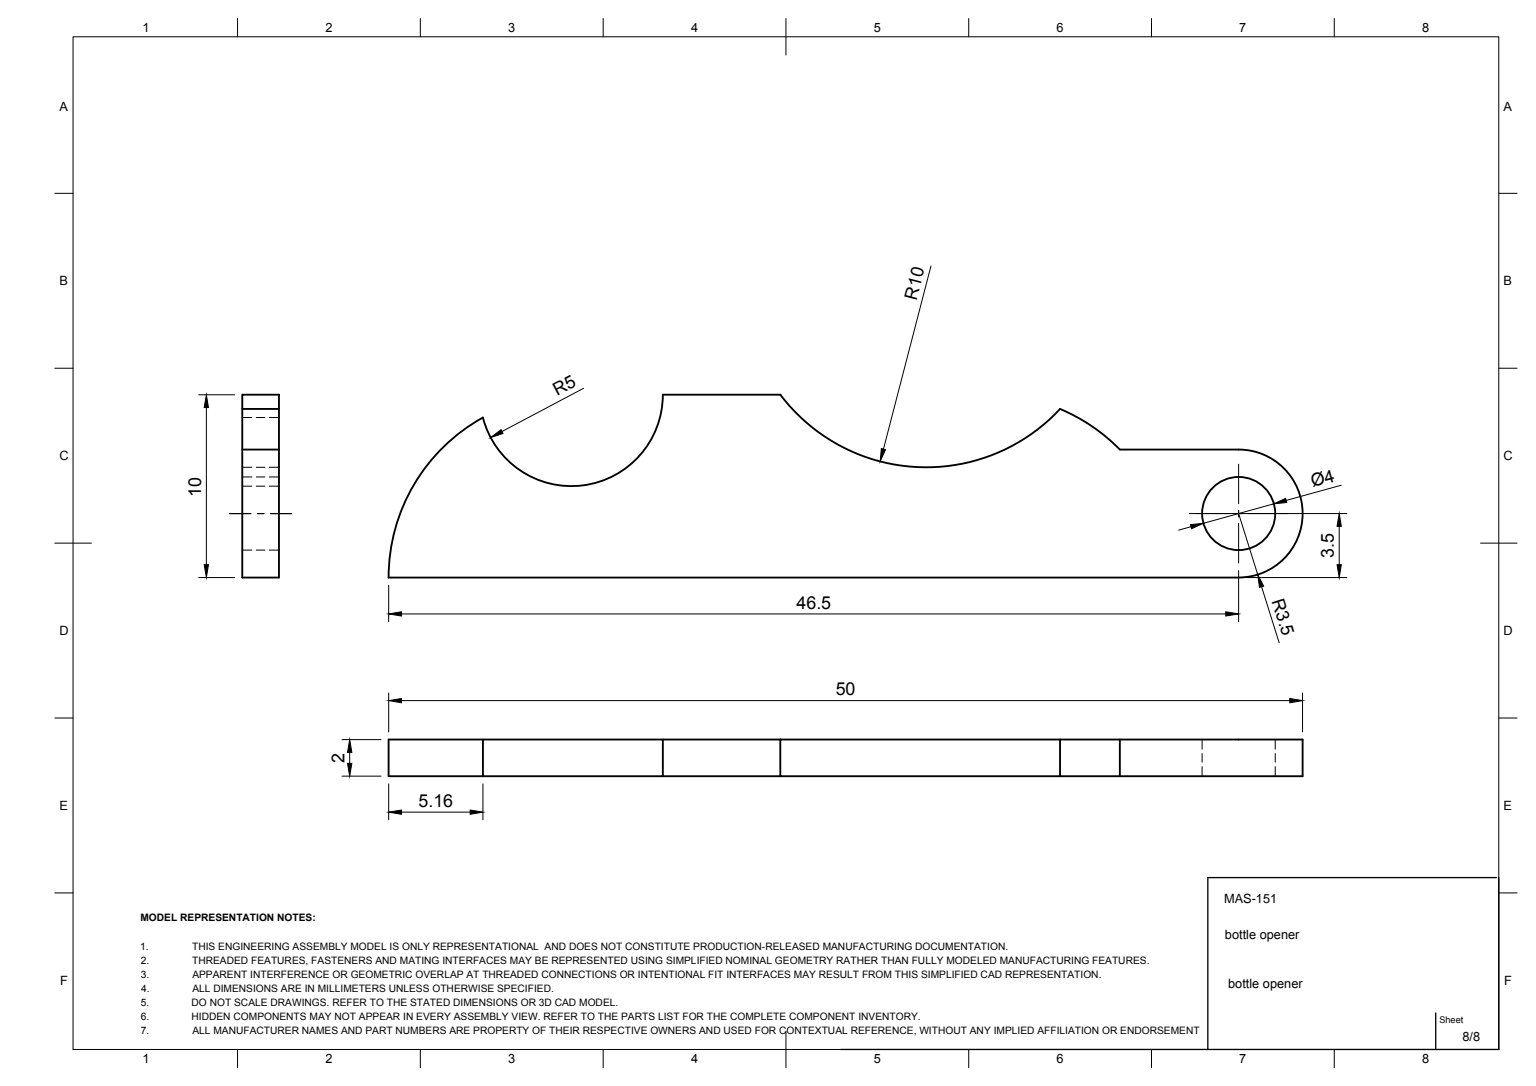
ISO-10303-21;
HEADER;
/* Generated by software containing ST-Developer
 * from STEP Tools, Inc. (www.steptools.com) 
 */

FILE_DESCRIPTION(
/* description */ ('STEP AP214'),
/* implementation_level */ '2;1');

FILE_NAME(
/* name */ 'bottle opener.step',
/* time_stamp */ '2026-11-04T19:14:12-08:00',
/* author */ (''),
/* organization */ (''),
/* preprocessor_version */ 'ST-DEVELOPER v20.2',
/* originating_system */ 'Autodesk Translation Framework v15.17.0.0',
/* authorisation */ '');

FILE_SCHEMA (('AUTOMOTIVE_DESIGN { 1 0 10303 214 3 1 1 }'));
ENDSEC;

DATA;
#10=MECHANICAL_DESIGN_GEOMETRIC_PRESENTATION_REPRESENTATION('',(#104),#5990);
#90=SHAPE_REPRESENTATION_RELATIONSHIP('SRR','None',#6026,#97);
#97=ADVANCED_BREP_SHAPE_REPRESENTATION('',(#111),#5988);
#104=STYLED_ITEM('',(#6068),#111);
#111=MANIFOLD_SOLID_BREP('Body1',#3274);
#133=FACE_BOUND('',#604,.T.);
#134=FACE_BOUND('',#606,.T.);
#233=PLANE('',#3648);
#234=PLANE('',#3652);
#235=PLANE('',#3656);
#236=PLANE('',#3657);
#237=PLANE('',#3658);
#402=FACE_OUTER_BOUND('',#600,.T.);
#403=FACE_OUTER_BOUND('',#601,.T.);
#404=FACE_OUTER_BOUND('',#602,.T.);
#405=FACE_OUTER_BOUND('',#603,.T.);
#406=FACE_OUTER_BOUND('',#605,.T.);
#407=FACE_OUTER_BOUND('',#607,.T.);
#408=FACE_OUTER_BOUND('',#608,.T.);
#409=FACE_OUTER_BOUND('',#609,.T.);
#410=FACE_OUTER_BOUND('',#610,.T.);
#411=FACE_OUTER_BOUND('',#611,.T.);
#412=FACE_OUTER_BOUND('',#612,.T.);
#600=EDGE_LOOP('',(#2956,#2957,#2958,#2959));
#601=EDGE_LOOP('',(#2960,#2961,#2962,#2963));
#602=EDGE_LOOP('',(#2964,#2965,#2966,#2967));
#603=EDGE_LOOP('',(#2968,#2969,#2970,#2971,#2972,#2973,#2974,#2975));
#604=EDGE_LOOP('',(#2976));
#605=EDGE_LOOP('',(#2977,#2978,#2979,#2980,#2981,#2982,#2983,#2984));
#606=EDGE_LOOP('',(#2985));
#607=EDGE_LOOP('',(#2986,#2987,#2988,#2989));
#608=EDGE_LOOP('',(#2990,#2991,#2992,#2993));
#609=EDGE_LOOP('',(#2994,#2995,#2996,#2997));
#610=EDGE_LOOP('',(#2998,#2999,#3000,#3001));
#611=EDGE_LOOP('',(#3002,#3003,#3004,#3005));
#612=EDGE_LOOP('',(#3006,#3007,#3008,#3009));
#907=LINE('',#5889,#1210);
#908=LINE('',#5896,#1211);
#909=LINE('',#5899,#1212);
#910=LINE('',#5905,#1213);
#911=LINE('',#5908,#1214);
#912=LINE('',#5912,#1215);
#913=LINE('',#5916,#1216);
#914=LINE('',#5918,#1217);
#915=LINE('',#5925,#1218);
#916=LINE('',#5927,#1219);
#917=LINE('',#5930,#1220);
#918=LINE('',#5933,#1221);
#919=LINE('',#5934,#1222);
#920=LINE('',#5936,#1223);
#921=LINE('',#5937,#1224);
#1210=VECTOR('',#4544,2.);
#1211=VECTOR('',#4551,1000.);
#1212=VECTOR('',#4554,1000.);
#1213=VECTOR('',#4559,1000.);
#1214=VECTOR('',#4562,1000.);
#1215=VECTOR('',#4565,1000.);
#1216=VECTOR('',#4568,1000.);
#1217=VECTOR('',#4571,1000.);
#1218=VECTOR('',#4578,1000.);
#1219=VECTOR('',#4581,1000.);
#1220=VECTOR('',#4584,1000.);
#1221=VECTOR('',#4589,1000.);
#1222=VECTOR('',#4590,1000.);
#1223=VECTOR('',#4593,1000.);
#1224=VECTOR('',#4594,1000.);
#1338=CIRCLE('',#3640,2.);
#1339=CIRCLE('',#3641,2.);
#1340=CIRCLE('',#3643,10.);
#1341=CIRCLE('',#3644,10.);
#1342=CIRCLE('',#3646,5.);
#1343=CIRCLE('',#3647,5.);
#1344=CIRCLE('',#3649,3.5);
#1345=CIRCLE('',#3650,10.);
#1346=CIRCLE('',#3651,10.);
#1347=CIRCLE('',#3653,3.5);
#1348=CIRCLE('',#3654,10.);
#1349=CIRCLE('',#3655,10.);
#1627=VERTEX_POINT('',#5886);
#1628=VERTEX_POINT('',#5888);
#1629=VERTEX_POINT('',#5892);
#1630=VERTEX_POINT('',#5893);
#1631=VERTEX_POINT('',#5895);
#1632=VERTEX_POINT('',#5897);
#1633=VERTEX_POINT('',#5901);
#1634=VERTEX_POINT('',#5902);
#1635=VERTEX_POINT('',#5904);
#1636=VERTEX_POINT('',#5906);
#1637=VERTEX_POINT('',#5910);
#1638=VERTEX_POINT('',#5911);
#1639=VERTEX_POINT('',#5913);
#1640=VERTEX_POINT('',#5915);
#1641=VERTEX_POINT('',#5921);
#1642=VERTEX_POINT('',#5922);
#1643=VERTEX_POINT('',#5924);
#1644=VERTEX_POINT('',#5928);
#2074=EDGE_CURVE('',#1627,#1627,#1338,.T.);
#2075=EDGE_CURVE('',#1627,#1628,#907,.T.);
#2076=EDGE_CURVE('',#1628,#1628,#1339,.T.);
#2077=EDGE_CURVE('',#1629,#1630,#1340,.T.);
#2078=EDGE_CURVE('',#1629,#1631,#908,.T.);
#2079=EDGE_CURVE('',#1631,#1632,#1341,.T.);
#2080=EDGE_CURVE('',#1630,#1632,#909,.T.);
#2081=EDGE_CURVE('',#1633,#1634,#1342,.T.);
#2082=EDGE_CURVE('',#1633,#1635,#910,.T.);
#2083=EDGE_CURVE('',#1635,#1636,#1343,.T.);
#2084=EDGE_CURVE('',#1636,#1634,#911,.T.);
#2085=EDGE_CURVE('',#1637,#1638,#912,.T.);
#2086=EDGE_CURVE('',#1637,#1639,#1344,.T.);
#2087=EDGE_CURVE('',#1639,#1640,#913,.T.);
#2088=EDGE_CURVE('',#1640,#1629,#1345,.T.);
#2089=EDGE_CURVE('',#1633,#1630,#914,.T.);
#2090=EDGE_CURVE('',#1634,#1638,#1346,.T.);
#2091=EDGE_CURVE('',#1641,#1642,#1347,.T.);
#2092=EDGE_CURVE('',#1642,#1643,#915,.T.);
#2093=EDGE_CURVE('',#1643,#1636,#1348,.T.);
#2094=EDGE_CURVE('',#1632,#1635,#916,.T.);
#2095=EDGE_CURVE('',#1631,#1644,#1349,.T.);
#2096=EDGE_CURVE('',#1641,#1644,#917,.T.);
#2097=EDGE_CURVE('',#1639,#1641,#918,.T.);
#2098=EDGE_CURVE('',#1640,#1644,#919,.T.);
#2099=EDGE_CURVE('',#1642,#1637,#920,.T.);
#2100=EDGE_CURVE('',#1638,#1643,#921,.T.);
#2956=ORIENTED_EDGE('',*,*,#2074,.F.);
#2957=ORIENTED_EDGE('',*,*,#2075,.T.);
#2958=ORIENTED_EDGE('',*,*,#2076,.F.);
#2959=ORIENTED_EDGE('',*,*,#2075,.F.);
#2960=ORIENTED_EDGE('',*,*,#2077,.F.);
#2961=ORIENTED_EDGE('',*,*,#2078,.T.);
#2962=ORIENTED_EDGE('',*,*,#2079,.T.);
#2963=ORIENTED_EDGE('',*,*,#2080,.F.);
#2964=ORIENTED_EDGE('',*,*,#2081,.F.);
#2965=ORIENTED_EDGE('',*,*,#2082,.T.);
#2966=ORIENTED_EDGE('',*,*,#2083,.T.);
#2967=ORIENTED_EDGE('',*,*,#2084,.T.);
#2968=ORIENTED_EDGE('',*,*,#2085,.F.);
#2969=ORIENTED_EDGE('',*,*,#2086,.T.);
#2970=ORIENTED_EDGE('',*,*,#2087,.T.);
#2971=ORIENTED_EDGE('',*,*,#2088,.T.);
#2972=ORIENTED_EDGE('',*,*,#2077,.T.);
#2973=ORIENTED_EDGE('',*,*,#2089,.F.);
#2974=ORIENTED_EDGE('',*,*,#2081,.T.);
#2975=ORIENTED_EDGE('',*,*,#2090,.T.);
#2976=ORIENTED_EDGE('',*,*,#2074,.T.);
#2977=ORIENTED_EDGE('',*,*,#2091,.T.);
#2978=ORIENTED_EDGE('',*,*,#2092,.T.);
#2979=ORIENTED_EDGE('',*,*,#2093,.T.);
#2980=ORIENTED_EDGE('',*,*,#2083,.F.);
#2981=ORIENTED_EDGE('',*,*,#2094,.F.);
#2982=ORIENTED_EDGE('',*,*,#2079,.F.);
#2983=ORIENTED_EDGE('',*,*,#2095,.T.);
#2984=ORIENTED_EDGE('',*,*,#2096,.F.);
#2985=ORIENTED_EDGE('',*,*,#2076,.T.);
#2986=ORIENTED_EDGE('',*,*,#2089,.T.);
#2987=ORIENTED_EDGE('',*,*,#2080,.T.);
#2988=ORIENTED_EDGE('',*,*,#2094,.T.);
#2989=ORIENTED_EDGE('',*,*,#2082,.F.);
#2990=ORIENTED_EDGE('',*,*,#2087,.F.);
#2991=ORIENTED_EDGE('',*,*,#2097,.T.);
#2992=ORIENTED_EDGE('',*,*,#2096,.T.);
#2993=ORIENTED_EDGE('',*,*,#2098,.F.);
#2994=ORIENTED_EDGE('',*,*,#2092,.F.);
#2995=ORIENTED_EDGE('',*,*,#2099,.T.);
#2996=ORIENTED_EDGE('',*,*,#2085,.T.);
#2997=ORIENTED_EDGE('',*,*,#2100,.T.);
#2998=ORIENTED_EDGE('',*,*,#2078,.F.);
#2999=ORIENTED_EDGE('',*,*,#2088,.F.);
#3000=ORIENTED_EDGE('',*,*,#2098,.T.);
#3001=ORIENTED_EDGE('',*,*,#2095,.F.);
#3002=ORIENTED_EDGE('',*,*,#2084,.F.);
#3003=ORIENTED_EDGE('',*,*,#2093,.F.);
#3004=ORIENTED_EDGE('',*,*,#2100,.F.);
#3005=ORIENTED_EDGE('',*,*,#2090,.F.);
#3006=ORIENTED_EDGE('',*,*,#2097,.F.);
#3007=ORIENTED_EDGE('',*,*,#2086,.F.);
#3008=ORIENTED_EDGE('',*,*,#2099,.F.);
#3009=ORIENTED_EDGE('',*,*,#2091,.F.);
#3082=CYLINDRICAL_SURFACE('',#3639,2.);
#3083=CYLINDRICAL_SURFACE('',#3642,10.);
#3084=CYLINDRICAL_SURFACE('',#3645,5.);
#3085=CYLINDRICAL_SURFACE('',#3659,10.);
#3086=CYLINDRICAL_SURFACE('',#3660,10.);
#3087=CYLINDRICAL_SURFACE('',#3661,3.5);
#3251=ADVANCED_FACE('',(#402),#3082,.F.);
#3252=ADVANCED_FACE('',(#403),#3083,.F.);
#3253=ADVANCED_FACE('',(#404),#3084,.F.);
#3254=ADVANCED_FACE('',(#405,#133),#233,.T.);
#3255=ADVANCED_FACE('',(#406,#134),#234,.F.);
#3256=ADVANCED_FACE('',(#407),#235,.T.);
#3257=ADVANCED_FACE('',(#408),#236,.F.);
#3258=ADVANCED_FACE('',(#409),#237,.T.);
#3259=ADVANCED_FACE('',(#410),#3085,.T.);
#3260=ADVANCED_FACE('',(#411),#3086,.T.);
#3261=ADVANCED_FACE('',(#412),#3087,.T.);
#3274=CLOSED_SHELL('',(#3251,#3252,#3253,#3254,#3255,#3256,#3257,#3258,
#3259,#3260,#3261));
#3638=AXIS2_PLACEMENT_3D('',#5884,#4538,#4539);
#3639=AXIS2_PLACEMENT_3D('',#5885,#4540,#4541);
#3640=AXIS2_PLACEMENT_3D('',#5887,#4542,#4543);
#3641=AXIS2_PLACEMENT_3D('',#5890,#4545,#4546);
#3642=AXIS2_PLACEMENT_3D('',#5891,#4547,#4548);
#3643=AXIS2_PLACEMENT_3D('',#5894,#4549,#4550);
#3644=AXIS2_PLACEMENT_3D('',#5898,#4552,#4553);
#3645=AXIS2_PLACEMENT_3D('',#5900,#4555,#4556);
#3646=AXIS2_PLACEMENT_3D('',#5903,#4557,#4558);
#3647=AXIS2_PLACEMENT_3D('',#5907,#4560,#4561);
#3648=AXIS2_PLACEMENT_3D('',#5909,#4563,#4564);
#3649=AXIS2_PLACEMENT_3D('',#5914,#4566,#4567);
#3650=AXIS2_PLACEMENT_3D('',#5917,#4569,#4570);
#3651=AXIS2_PLACEMENT_3D('',#5919,#4572,#4573);
#3652=AXIS2_PLACEMENT_3D('',#5920,#4574,#4575);
#3653=AXIS2_PLACEMENT_3D('',#5923,#4576,#4577);
#3654=AXIS2_PLACEMENT_3D('',#5926,#4579,#4580);
#3655=AXIS2_PLACEMENT_3D('',#5929,#4582,#4583);
#3656=AXIS2_PLACEMENT_3D('',#5931,#4585,#4586);
#3657=AXIS2_PLACEMENT_3D('',#5932,#4587,#4588);
#3658=AXIS2_PLACEMENT_3D('',#5935,#4591,#4592);
#3659=AXIS2_PLACEMENT_3D('',#5938,#4595,#4596);
#3660=AXIS2_PLACEMENT_3D('',#5939,#4597,#4598);
#3661=AXIS2_PLACEMENT_3D('',#5940,#4599,#4600);
#4538=DIRECTION('axis',(0.,0.,1.));
#4539=DIRECTION('refdir',(1.,0.,0.));
#4540=DIRECTION('center_axis',(0.,6.83705130257469E-33,1.));
#4541=DIRECTION('ref_axis',(1.,0.,0.));
#4542=DIRECTION('center_axis',(-1.34131666839389E-70,6.83705130257469E-33,
1.));
#4543=DIRECTION('ref_axis',(1.,0.,0.));
#4544=DIRECTION('',(0.,6.83705130257469E-33,1.));
#4545=DIRECTION('center_axis',(0.,-6.83705130257469E-33,-1.));
#4546=DIRECTION('ref_axis',(-1.,0.,0.));
#4547=DIRECTION('center_axis',(0.,6.83705130257469E-33,1.));
#4548=DIRECTION('ref_axis',(1.,0.,0.));
#4549=DIRECTION('center_axis',(0.,6.83705130257469E-33,1.));
#4550=DIRECTION('ref_axis',(1.,0.,0.));
#4551=DIRECTION('',(0.,6.83705130257469E-33,1.));
#4552=DIRECTION('center_axis',(-1.34131666839389E-70,6.83705130257469E-33,
1.));
#4553=DIRECTION('ref_axis',(1.,0.,0.));
#4554=DIRECTION('',(0.,6.83705130257469E-33,1.));
#4555=DIRECTION('center_axis',(0.,6.83705130257469E-33,1.));
#4556=DIRECTION('ref_axis',(1.,0.,0.));
#4557=DIRECTION('center_axis',(0.,6.83705130257469E-33,1.));
#4558=DIRECTION('ref_axis',(1.,0.,0.));
#4559=DIRECTION('',(0.,6.83705130257469E-33,1.));
#4560=DIRECTION('center_axis',(-1.34131666839389E-70,6.83705130257469E-33,
1.));
#4561=DIRECTION('ref_axis',(1.,0.,0.));
#4562=DIRECTION('',(0.,-6.83705130257469E-33,-1.));
#4563=DIRECTION('center_axis',(1.34131666839389E-70,-6.83705130257469E-33,
-1.));
#4564=DIRECTION('ref_axis',(-1.,-1.96183502073295E-38,0.));
#4565=DIRECTION('',(1.96183502073296E-38,1.,6.83705130257469E-33));
#4566=DIRECTION('center_axis',(0.,-6.83705130257469E-33,-1.));
#4567=DIRECTION('ref_axis',(-1.,0.,0.));
#4568=DIRECTION('',(1.96183502073296E-38,1.,6.83705130257469E-33));
#4569=DIRECTION('center_axis',(0.,-6.83705130257469E-33,-1.));
#4570=DIRECTION('ref_axis',(-1.,0.,0.));
#4571=DIRECTION('',(-1.96183502143475E-38,-1.,1.19262238973405E-16));
#4572=DIRECTION('center_axis',(0.,-6.83705130257469E-33,-1.));
#4573=DIRECTION('ref_axis',(-1.,0.,0.));
#4574=DIRECTION('center_axis',(1.34131666839389E-70,-6.83705130257469E-33,
-1.));
#4575=DIRECTION('ref_axis',(-1.,-1.96183502073295E-38,0.));
#4576=DIRECTION('center_axis',(0.,6.83705130257469E-33,1.));
#4577=DIRECTION('ref_axis',(-1.,0.,0.));
#4578=DIRECTION('',(1.96183502073296E-38,1.,6.83705130257469E-33));
#4579=DIRECTION('center_axis',(0.,6.83705130257469E-33,1.));
#4580=DIRECTION('ref_axis',(-1.,0.,0.));
#4581=DIRECTION('',(1.96183502073296E-38,1.,6.83705130257469E-33));
#4582=DIRECTION('center_axis',(0.,6.83705130257469E-33,1.));
#4583=DIRECTION('ref_axis',(-1.,1.38777878078145E-15,-9.4883147208273E-48));
#4584=DIRECTION('',(1.96183502073296E-38,1.,6.83705130257469E-33));
#4585=DIRECTION('center_axis',(-1.,-1.96183502073295E-38,1.34131666839389E-70));
#4586=DIRECTION('ref_axis',(0.,6.83705130257469E-33,1.));
#4587=DIRECTION('center_axis',(1.,1.96183502073295E-38,-1.34131666839389E-70));
#4588=DIRECTION('ref_axis',(0.,-6.83705130257469E-33,-1.));
#4589=DIRECTION('',(0.,6.83705130257469E-33,1.));
#4590=DIRECTION('',(0.,6.83705130257469E-33,1.));
#4591=DIRECTION('center_axis',(1.,1.96183502073295E-38,-1.34131666839389E-70));
#4592=DIRECTION('ref_axis',(0.,-6.83705130257469E-33,-1.));
#4593=DIRECTION('',(0.,-6.83705130257469E-33,-1.));
#4594=DIRECTION('',(0.,6.83705130257469E-33,1.));
#4595=DIRECTION('center_axis',(0.,-6.83705130257469E-33,-1.));
#4596=DIRECTION('ref_axis',(-1.,0.,0.));
#4597=DIRECTION('center_axis',(0.,6.83705130257469E-33,1.));
#4598=DIRECTION('ref_axis',(1.,0.,0.));
#4599=DIRECTION('center_axis',(0.,6.83705130257469E-33,1.));
#4600=DIRECTION('ref_axis',(1.,0.,0.));
#5884=CARTESIAN_POINT('',(0.,0.,0.));
#5885=CARTESIAN_POINT('Origin',(-16.,-116.5,-2.000025));
#5886=CARTESIAN_POINT('',(-18.,-116.5,-2.));
#5887=CARTESIAN_POINT('Origin',(-16.,-116.5,-2.));
#5888=CARTESIAN_POINT('',(-18.,-116.5,0.));
#5889=CARTESIAN_POINT('',(-18.,-116.5,-2.000025));
#5890=CARTESIAN_POINT('Origin',(-16.,-116.5,-3.05741378671474E-30));
#5891=CARTESIAN_POINT('Origin',(-28.5285484527122,-99.4077946409786,-1.99999999999999));
#5892=CARTESIAN_POINT('',(-21.7195444572929,-106.731554917665,-1.99999999999999));
#5893=CARTESIAN_POINT('',(-22.5,-91.4292857857286,-1.99999999999999));
#5894=CARTESIAN_POINT('Origin',(-28.5285484527122,-99.4077946409786,-1.99999999999999));
#5895=CARTESIAN_POINT('',(-21.7195444572929,-106.731554917665,6.01457402401214E-10));
#5896=CARTESIAN_POINT('',(-21.7195444572929,-106.731554917665,-1.99999999999999));
#5897=CARTESIAN_POINT('',(-22.5,-91.4292857857286,2.40741243048404E-32));
#5898=CARTESIAN_POINT('Origin',(-28.5285484527122,-99.4077946409786,0.));
#5899=CARTESIAN_POINT('',(-22.5,-91.4292857857286,-1.99999999999999));
#5900=CARTESIAN_POINT('Origin',(-22.5,-80.0000000000001,-1.99999999999999));
#5901=CARTESIAN_POINT('',(-22.5,-85.0000000000001,-1.99999999999999));
#5902=CARTESIAN_POINT('',(-21.25,-75.1587708172408,-2.));
#5903=CARTESIAN_POINT('Origin',(-22.5,-80.0000000000001,-1.99999999999999));
#5904=CARTESIAN_POINT('',(-22.4999999999998,-85.0000000000001,6.01457402401214E-10));
#5905=CARTESIAN_POINT('',(-22.5,-85.0000000000001,-1.99999999999999));
#5906=CARTESIAN_POINT('',(-21.2500000008195,-75.1587708175933,8.25034485174569E-13));
#5907=CARTESIAN_POINT('Origin',(-22.5,-80.0000000000001,0.));
#5908=CARTESIAN_POINT('',(-21.25,-75.1587708172408,-0.999994));
#5909=CARTESIAN_POINT('Origin',(0.,0.,-2.));
#5910=CARTESIAN_POINT('',(-12.5,-116.5,-2.));
#5911=CARTESIAN_POINT('',(-12.5,-70.,-2.));
#5912=CARTESIAN_POINT('',(-12.5,-120.,-2.));
#5913=CARTESIAN_POINT('',(-19.5,-116.5,-2.));
#5914=CARTESIAN_POINT('Origin',(-16.,-116.5,-2.));
#5915=CARTESIAN_POINT('',(-19.5,-110.,-2.));
#5916=CARTESIAN_POINT('',(-19.5,-120.,-2.));
#5917=CARTESIAN_POINT('Origin',(-12.5,-102.858571571457,-2.));
#5918=CARTESIAN_POINT('',(-22.5,-70.,-1.99999999999999));
#5919=CARTESIAN_POINT('Origin',(-12.5,-80.,-2.));
#5920=CARTESIAN_POINT('Origin',(0.,0.,0.));
#5921=CARTESIAN_POINT('',(-19.5,-116.5,-3.05741378671474E-30));
#5922=CARTESIAN_POINT('',(-12.5,-116.5,-7.22223729145213E-32));
#5923=CARTESIAN_POINT('Origin',(-16.,-116.5,-3.1537102839341E-30));
#5924=CARTESIAN_POINT('',(-12.5,-70.,-7.22223729145213E-32));
#5925=CARTESIAN_POINT('',(-12.5,-120.,-3.05741378671474E-30));
#5926=CARTESIAN_POINT('Origin',(-12.5,-80.,-7.22223729145213E-32));
#5927=CARTESIAN_POINT('',(-22.5,-70.,-3.05741378671474E-30));
#5928=CARTESIAN_POINT('',(-19.5,-110.,-7.22223729145213E-32));
#5929=CARTESIAN_POINT('Origin',(-12.5,-102.858571571457,-7.22223729145213E-32));
#5930=CARTESIAN_POINT('',(-19.5,-120.,-3.1537102839341E-30));
#5931=CARTESIAN_POINT('Origin',(-22.5,0.,2.40741243048404E-32));
#5932=CARTESIAN_POINT('Origin',(-19.5,-120.,-2.));
#5933=CARTESIAN_POINT('',(-19.5,-116.5,-2.));
#5934=CARTESIAN_POINT('',(-19.5,-110.,-2.));
#5935=CARTESIAN_POINT('Origin',(-12.5,-120.,-2.));
#5936=CARTESIAN_POINT('',(-12.5,-116.5,-2.));
#5937=CARTESIAN_POINT('',(-12.5,-70.,-2.));
#5938=CARTESIAN_POINT('Origin',(-12.5,-102.858571571457,-2.));
#5939=CARTESIAN_POINT('Origin',(-12.5,-80.,-7.22223729145213E-32));
#5940=CARTESIAN_POINT('Origin',(-16.,-116.5,-2.));
#5979=UNCERTAINTY_MEASURE_WITH_UNIT(LENGTH_MEASURE(0.01),#5991,
'DISTANCE_ACCURACY_VALUE',
'Maximum model space distance between geometric entities at asserted c
onnectivities');
#5981=UNCERTAINTY_MEASURE_WITH_UNIT(LENGTH_MEASURE(0.01),#5991,
'DISTANCE_ACCURACY_VALUE',
'Maximum model space distance between geometric entities at asserted c
onnectivities');
#5988=(
GEOMETRIC_REPRESENTATION_CONTEXT(3)
GLOBAL_UNCERTAINTY_ASSIGNED_CONTEXT((#5979))
GLOBAL_UNIT_ASSIGNED_CONTEXT((#5991,#5993,#5994))
REPRESENTATION_CONTEXT('','3D')
);
#5990=(
GEOMETRIC_REPRESENTATION_CONTEXT(3)
GLOBAL_UNCERTAINTY_ASSIGNED_CONTEXT((#5981))
GLOBAL_UNIT_ASSIGNED_CONTEXT((#5991,#5993,#5994))
REPRESENTATION_CONTEXT('','3D')
);
#5991=(
LENGTH_UNIT()
NAMED_UNIT(*)
SI_UNIT(.MILLI.,.METRE.)
);
#5993=(
NAMED_UNIT(*)
PLANE_ANGLE_UNIT()
SI_UNIT($,.RADIAN.)
);
#5994=(
NAMED_UNIT(*)
SI_UNIT($,.STERADIAN.)
SOLID_ANGLE_UNIT()
);
#6001=SHAPE_DEFINITION_REPRESENTATION(#6009,#6026);
#6009=PRODUCT_DEFINITION_SHAPE('',$,#6035);
#6026=SHAPE_REPRESENTATION('',(#3638),#5988);
#6028=PRODUCT_DEFINITION_CONTEXT('part definition',#6054,'design');
#6035=PRODUCT_DEFINITION('bottle opener','bottle opener',#6043,#6028);
#6043=PRODUCT_DEFINITION_FORMATION('',$,#6062);
#6054=APPLICATION_CONTEXT(
'Core Data for Automotive Mechanical Design Process');
#6055=PRODUCT_CONTEXT('part definition',#6054,'mechanical');
#6062=PRODUCT('bottle opener','bottle opener',$,(#6055));
#6068=PRESENTATION_STYLE_ASSIGNMENT((#6074));
#6074=SURFACE_STYLE_USAGE(.BOTH.,#6080);
#6080=SURFACE_SIDE_STYLE('',(#6086));
#6086=SURFACE_STYLE_FILL_AREA(#6092);
#6092=FILL_AREA_STYLE('Opaque(227,224,212)',(#6098));
#6098=FILL_AREA_STYLE_COLOUR('Opaque(227,224,212)',#6104);
#6104=COLOUR_RGB('Opaque(227,224,212)',0.890196078431372,0.87843137254902,
0.831372549019608);
ENDSEC;
END-ISO-10303-21;
